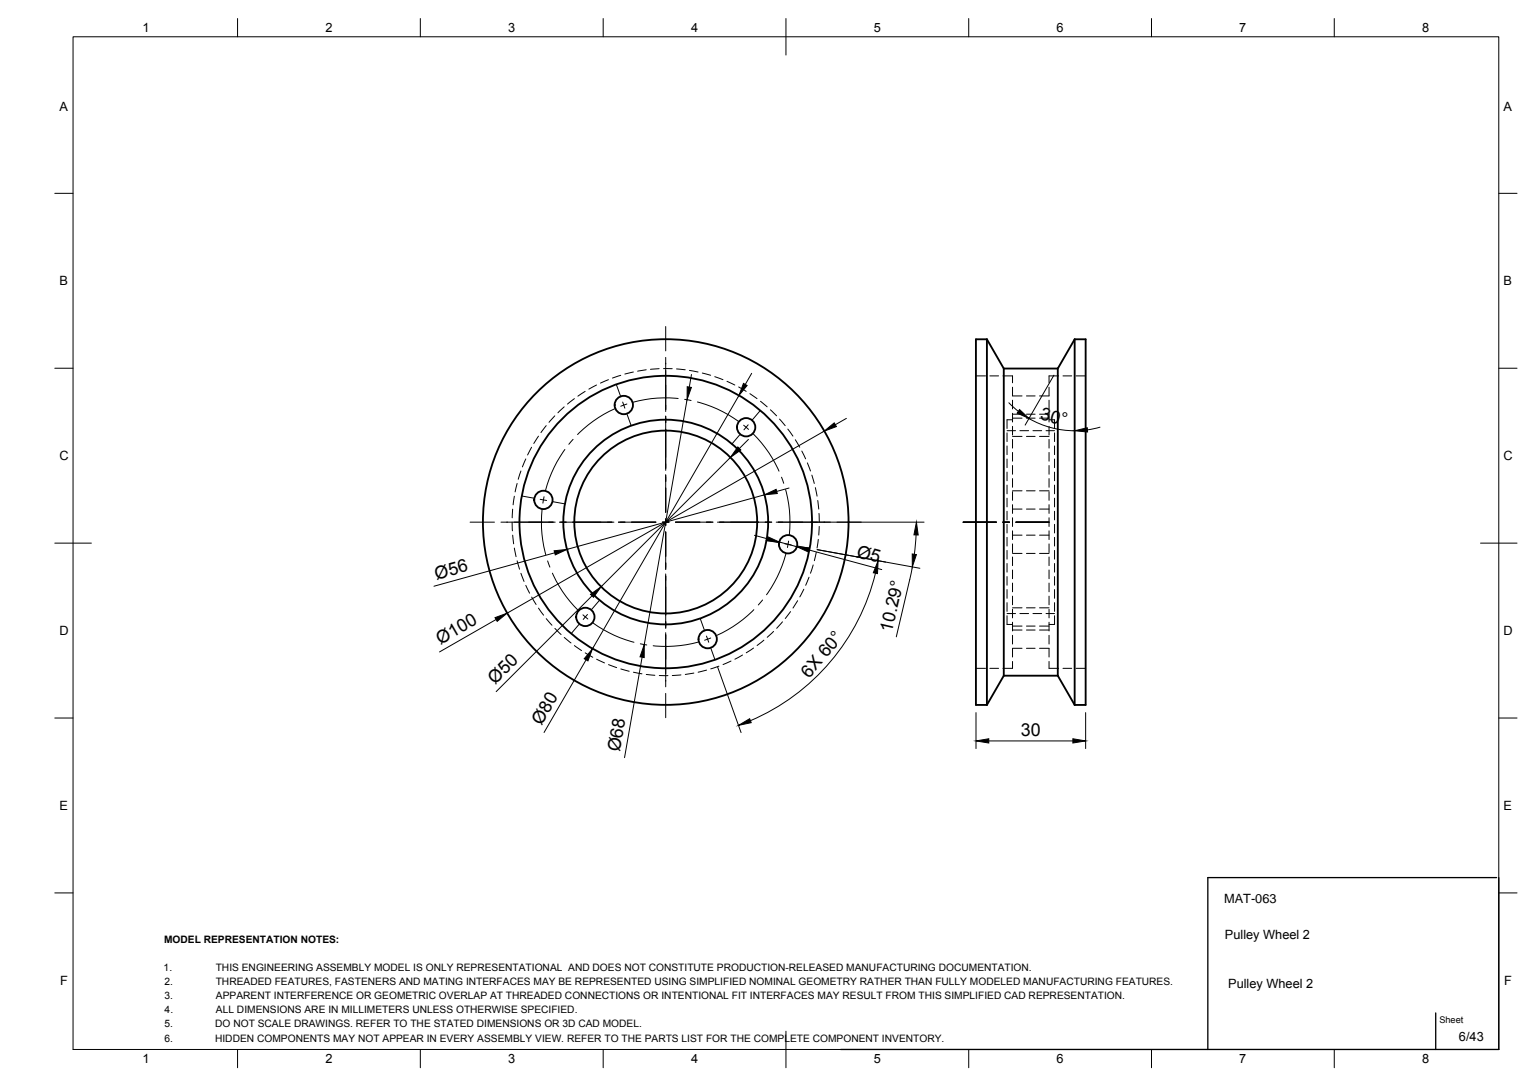
ISO-10303-21;
HEADER;
/* Generated by software containing ST-Developer
 * from STEP Tools, Inc. (www.steptools.com) 
 */

FILE_DESCRIPTION(
/* description */ (''),
/* implementation_level */ '2;1');

FILE_NAME(
/* name */ 'Pulley Wheel 2.step',
/* time_stamp */ '2026-10-24T09:43:01-07:00',
/* author */ (''),
/* organization */ (''),
/* preprocessor_version */ 'ST-DEVELOPER v20.2',
/* originating_system */ 'Autodesk Translation Framework v15.15.0.0',
/* authorisation */ '');

FILE_SCHEMA (('AUTOMOTIVE_DESIGN { 1 0 10303 214 3 1 1 }'));
ENDSEC;

DATA;
#10=MECHANICAL_DESIGN_GEOMETRIC_PRESENTATION_REPRESENTATION('',(#276),#11112);
#210=SHAPE_REPRESENTATION_RELATIONSHIP('SRR','None',#11233,#243);
#243=ADVANCED_BREP_SHAPE_REPRESENTATION('',(#309),#11078);
#276=STYLED_ITEM('',(#11424),#309);
#309=MANIFOLD_SOLID_BREP('Pulley Wheel 2',#6013);
#365=FACE_BOUND('',#1131,.T.);
#366=FACE_BOUND('',#1133,.T.);
#367=FACE_BOUND('',#1137,.T.);
#368=FACE_BOUND('',#1138,.T.);
#369=FACE_BOUND('',#1139,.T.);
#370=FACE_BOUND('',#1140,.T.);
#371=FACE_BOUND('',#1141,.T.);
#372=FACE_BOUND('',#1142,.T.);
#373=FACE_BOUND('',#1143,.T.);
#374=FACE_BOUND('',#1145,.T.);
#375=FACE_BOUND('',#1146,.T.);
#376=FACE_BOUND('',#1147,.T.);
#377=FACE_BOUND('',#1148,.T.);
#378=FACE_BOUND('',#1149,.T.);
#379=FACE_BOUND('',#1150,.T.);
#380=FACE_BOUND('',#1151,.T.);
#381=FACE_BOUND('',#1161,.T.);
#382=FACE_BOUND('',#1163,.T.);
#510=PLANE('',#6593);
#511=PLANE('',#6595);
#512=PLANE('',#6601);
#513=PLANE('',#6609);
#514=PLANE('',#6627);
#515=PLANE('',#6629);
#667=CONICAL_SURFACE('',#6584,1.,1.04719756558882);
#668=CONICAL_SURFACE('',#6586,1.,1.04719756558882);
#735=FACE_OUTER_BOUND('',#1125,.T.);
#736=FACE_OUTER_BOUND('',#1126,.T.);
#737=FACE_OUTER_BOUND('',#1127,.T.);
#738=FACE_OUTER_BOUND('',#1128,.T.);
#739=FACE_OUTER_BOUND('',#1129,.T.);
#740=FACE_OUTER_BOUND('',#1130,.T.);
#741=FACE_OUTER_BOUND('',#1132,.T.);
#742=FACE_OUTER_BOUND('',#1134,.T.);
#743=FACE_OUTER_BOUND('',#1135,.T.);
#744=FACE_OUTER_BOUND('',#1136,.T.);
#745=FACE_OUTER_BOUND('',#1144,.T.);
#746=FACE_OUTER_BOUND('',#1152,.T.);
#747=FACE_OUTER_BOUND('',#1153,.T.);
#748=FACE_OUTER_BOUND('',#1154,.T.);
#749=FACE_OUTER_BOUND('',#1155,.T.);
#750=FACE_OUTER_BOUND('',#1156,.T.);
#751=FACE_OUTER_BOUND('',#1157,.T.);
#752=FACE_OUTER_BOUND('',#1158,.T.);
#753=FACE_OUTER_BOUND('',#1159,.T.);
#754=FACE_OUTER_BOUND('',#1160,.T.);
#755=FACE_OUTER_BOUND('',#1162,.T.);
#756=FACE_OUTER_BOUND('',#1164,.T.);
#1125=EDGE_LOOP('',(#4221,#4222,#4223,#4224,#4225));
#1126=EDGE_LOOP('',(#4226,#4227,#4228,#4229,#4230));
#1127=EDGE_LOOP('',(#4231,#4232,#4233,#4234,#4235));
#1128=EDGE_LOOP('',(#4236,#4237,#4238,#4239));
#1129=EDGE_LOOP('',(#4240,#4241,#4242,#4243,#4244));
#1130=EDGE_LOOP('',(#4245));
#1131=EDGE_LOOP('',(#4246));
#1132=EDGE_LOOP('',(#4247));
#1133=EDGE_LOOP('',(#4248));
#1134=EDGE_LOOP('',(#4249,#4250,#4251,#4252));
#1135=EDGE_LOOP('',(#4253,#4254,#4255,#4256));
#1136=EDGE_LOOP('',(#4257));
#1137=EDGE_LOOP('',(#4258));
#1138=EDGE_LOOP('',(#4259));
#1139=EDGE_LOOP('',(#4260));
#1140=EDGE_LOOP('',(#4261));
#1141=EDGE_LOOP('',(#4262));
#1142=EDGE_LOOP('',(#4263));
#1143=EDGE_LOOP('',(#4264));
#1144=EDGE_LOOP('',(#4265));
#1145=EDGE_LOOP('',(#4266));
#1146=EDGE_LOOP('',(#4267));
#1147=EDGE_LOOP('',(#4268));
#1148=EDGE_LOOP('',(#4269));
#1149=EDGE_LOOP('',(#4270));
#1150=EDGE_LOOP('',(#4271));
#1151=EDGE_LOOP('',(#4272));
#1152=EDGE_LOOP('',(#4273,#4274,#4275,#4276));
#1153=EDGE_LOOP('',(#4277,#4278,#4279,#4280));
#1154=EDGE_LOOP('',(#4281,#4282,#4283,#4284));
#1155=EDGE_LOOP('',(#4285,#4286,#4287,#4288));
#1156=EDGE_LOOP('',(#4289,#4290,#4291,#4292));
#1157=EDGE_LOOP('',(#4293,#4294,#4295,#4296));
#1158=EDGE_LOOP('',(#4297,#4298,#4299,#4300));
#1159=EDGE_LOOP('',(#4301,#4302,#4303,#4304));
#1160=EDGE_LOOP('',(#4305));
#1161=EDGE_LOOP('',(#4306));
#1162=EDGE_LOOP('',(#4307));
#1163=EDGE_LOOP('',(#4308));
#1164=EDGE_LOOP('',(#4309,#4310,#4311,#4312));
#1586=LINE('',#9616,#1945);
#1587=LINE('',#9623,#1946);
#1588=LINE('',#9628,#1947);
#1589=LINE('',#9633,#1948);
#1590=LINE('',#9636,#1949);
#1591=LINE('',#9647,#1950);
#1592=LINE('',#9650,#1951);
#1593=LINE('',#9685,#1952);
#1594=LINE('',#9687,#1953);
#1595=LINE('',#9689,#1954);
#1596=LINE('',#9691,#1955);
#1597=LINE('',#9693,#1956);
#1598=LINE('',#9695,#1957);
#1599=LINE('',#9697,#1958);
#1600=LINE('',#9700,#1959);
#1601=LINE('',#9709,#1960);
#1945=VECTOR('',#7638,0.042);
#1946=VECTOR('',#7647,1.);
#1947=VECTOR('',#7652,1.);
#1948=VECTOR('',#7659,0.05);
#1949=VECTOR('',#7662,0.05);
#1950=VECTOR('',#7677,0.04);
#1951=VECTOR('',#7680,0.04);
#1952=VECTOR('',#7719,0.028);
#1953=VECTOR('',#7722,0.0025);
#1954=VECTOR('',#7725,0.0025);
#1955=VECTOR('',#7728,0.0025);
#1956=VECTOR('',#7731,0.0025);
#1957=VECTOR('',#7734,0.0025);
#1958=VECTOR('',#7737,0.0025);
#1959=VECTOR('',#7740,0.028);
#1960=VECTOR('',#7753,0.025);
#2382=CIRCLE('',#6581,0.042);
#2383=CIRCLE('',#6582,0.042);
#2384=CIRCLE('',#6583,0.042);
#2385=CIRCLE('',#6585,0.05);
#2386=CIRCLE('',#6587,0.05);
#2387=CIRCLE('',#6588,0.05);
#2388=CIRCLE('',#6590,0.05);
#2389=CIRCLE('',#6592,0.05);
#2390=CIRCLE('',#6594,0.04);
#2391=CIRCLE('',#6596,0.04);
#2392=CIRCLE('',#6598,0.04);
#2393=CIRCLE('',#6600,0.04);
#2394=CIRCLE('',#6602,0.0025);
#2395=CIRCLE('',#6603,0.0025);
#2396=CIRCLE('',#6604,0.0025);
#2397=CIRCLE('',#6605,0.0025);
#2398=CIRCLE('',#6606,0.0025);
#2399=CIRCLE('',#6607,0.0025);
#2400=CIRCLE('',#6608,0.028);
#2401=CIRCLE('',#6610,0.0025);
#2402=CIRCLE('',#6611,0.0025);
#2403=CIRCLE('',#6612,0.0025);
#2404=CIRCLE('',#6613,0.0025);
#2405=CIRCLE('',#6614,0.0025);
#2406=CIRCLE('',#6615,0.0025);
#2407=CIRCLE('',#6616,0.028);
#2408=CIRCLE('',#6618,0.028);
#2409=CIRCLE('',#6626,0.028);
#2410=CIRCLE('',#6628,0.025);
#2411=CIRCLE('',#6630,0.025);
#2768=VERTEX_POINT('',#9613);
#2769=VERTEX_POINT('',#9615);
#2770=VERTEX_POINT('',#9617);
#2771=VERTEX_POINT('',#9621);
#2772=VERTEX_POINT('',#9625);
#2773=VERTEX_POINT('',#9626);
#2774=VERTEX_POINT('',#9631);
#2775=VERTEX_POINT('',#9635);
#2776=VERTEX_POINT('',#9639);
#2777=VERTEX_POINT('',#9642);
#2778=VERTEX_POINT('',#9645);
#2779=VERTEX_POINT('',#9649);
#2780=VERTEX_POINT('',#9653);
#2781=VERTEX_POINT('',#9655);
#2782=VERTEX_POINT('',#9657);
#2783=VERTEX_POINT('',#9659);
#2784=VERTEX_POINT('',#9661);
#2785=VERTEX_POINT('',#9663);
#2786=VERTEX_POINT('',#9665);
#2787=VERTEX_POINT('',#9668);
#2788=VERTEX_POINT('',#9670);
#2789=VERTEX_POINT('',#9672);
#2790=VERTEX_POINT('',#9674);
#2791=VERTEX_POINT('',#9676);
#2792=VERTEX_POINT('',#9678);
#2793=VERTEX_POINT('',#9680);
#2794=VERTEX_POINT('',#9683);
#2795=VERTEX_POINT('',#9699);
#2796=VERTEX_POINT('',#9703);
#2797=VERTEX_POINT('',#9706);
#3314=EDGE_CURVE('',#2768,#2768,#2382,.F.);
#3315=EDGE_CURVE('',#2768,#2769,#1586,.T.);
#3316=EDGE_CURVE('',#2769,#2770,#2383,.F.);
#3317=EDGE_CURVE('',#2770,#2769,#2384,.F.);
#3318=EDGE_CURVE('',#2771,#2771,#2385,.F.);
#3319=EDGE_CURVE('',#2771,#2770,#1587,.T.);
#3320=EDGE_CURVE('',#2772,#2773,#2386,.F.);
#3321=EDGE_CURVE('',#2773,#2768,#1588,.T.);
#3322=EDGE_CURVE('',#2773,#2772,#2387,.F.);
#3323=EDGE_CURVE('',#2774,#2774,#2388,.F.);
#3324=EDGE_CURVE('',#2774,#2771,#1589,.T.);
#3325=EDGE_CURVE('',#2772,#2775,#1590,.T.);
#3326=EDGE_CURVE('',#2775,#2775,#2389,.T.);
#3327=EDGE_CURVE('',#2776,#2776,#2390,.T.);
#3328=EDGE_CURVE('',#2777,#2777,#2391,.T.);
#3329=EDGE_CURVE('',#2778,#2778,#2392,.T.);
#3330=EDGE_CURVE('',#2778,#2776,#1591,.T.);
#3331=EDGE_CURVE('',#2777,#2779,#1592,.T.);
#3332=EDGE_CURVE('',#2779,#2779,#2393,.F.);
#3333=EDGE_CURVE('',#2780,#2780,#2394,.F.);
#3334=EDGE_CURVE('',#2781,#2781,#2395,.F.);
#3335=EDGE_CURVE('',#2782,#2782,#2396,.F.);
#3336=EDGE_CURVE('',#2783,#2783,#2397,.F.);
#3337=EDGE_CURVE('',#2784,#2784,#2398,.F.);
#3338=EDGE_CURVE('',#2785,#2785,#2399,.F.);
#3339=EDGE_CURVE('',#2786,#2786,#2400,.T.);
#3340=EDGE_CURVE('',#2787,#2787,#2401,.F.);
#3341=EDGE_CURVE('',#2788,#2788,#2402,.F.);
#3342=EDGE_CURVE('',#2789,#2789,#2403,.F.);
#3343=EDGE_CURVE('',#2790,#2790,#2404,.F.);
#3344=EDGE_CURVE('',#2791,#2791,#2405,.F.);
#3345=EDGE_CURVE('',#2792,#2792,#2406,.F.);
#3346=EDGE_CURVE('',#2793,#2793,#2407,.T.);
#3347=EDGE_CURVE('',#2794,#2794,#2408,.F.);
#3348=EDGE_CURVE('',#2794,#2786,#1593,.T.);
#3349=EDGE_CURVE('',#2785,#2792,#1594,.T.);
#3350=EDGE_CURVE('',#2784,#2791,#1595,.T.);
#3351=EDGE_CURVE('',#2783,#2790,#1596,.T.);
#3352=EDGE_CURVE('',#2782,#2789,#1597,.T.);
#3353=EDGE_CURVE('',#2781,#2788,#1598,.T.);
#3354=EDGE_CURVE('',#2780,#2787,#1599,.T.);
#3355=EDGE_CURVE('',#2793,#2795,#1600,.T.);
#3356=EDGE_CURVE('',#2795,#2795,#2409,.T.);
#3357=EDGE_CURVE('',#2796,#2796,#2410,.T.);
#3358=EDGE_CURVE('',#2797,#2797,#2411,.T.);
#3359=EDGE_CURVE('',#2797,#2796,#1601,.T.);
#4221=ORIENTED_EDGE('',*,*,#3314,.T.);
#4222=ORIENTED_EDGE('',*,*,#3315,.T.);
#4223=ORIENTED_EDGE('',*,*,#3316,.T.);
#4224=ORIENTED_EDGE('',*,*,#3317,.T.);
#4225=ORIENTED_EDGE('',*,*,#3315,.F.);
#4226=ORIENTED_EDGE('',*,*,#3318,.T.);
#4227=ORIENTED_EDGE('',*,*,#3319,.T.);
#4228=ORIENTED_EDGE('',*,*,#3316,.F.);
#4229=ORIENTED_EDGE('',*,*,#3317,.F.);
#4230=ORIENTED_EDGE('',*,*,#3319,.F.);
#4231=ORIENTED_EDGE('',*,*,#3320,.T.);
#4232=ORIENTED_EDGE('',*,*,#3321,.T.);
#4233=ORIENTED_EDGE('',*,*,#3314,.F.);
#4234=ORIENTED_EDGE('',*,*,#3321,.F.);
#4235=ORIENTED_EDGE('',*,*,#3322,.T.);
#4236=ORIENTED_EDGE('',*,*,#3323,.T.);
#4237=ORIENTED_EDGE('',*,*,#3324,.T.);
#4238=ORIENTED_EDGE('',*,*,#3318,.F.);
#4239=ORIENTED_EDGE('',*,*,#3324,.F.);
#4240=ORIENTED_EDGE('',*,*,#3320,.F.);
#4241=ORIENTED_EDGE('',*,*,#3325,.T.);
#4242=ORIENTED_EDGE('',*,*,#3326,.T.);
#4243=ORIENTED_EDGE('',*,*,#3325,.F.);
#4244=ORIENTED_EDGE('',*,*,#3322,.F.);
#4245=ORIENTED_EDGE('',*,*,#3323,.F.);
#4246=ORIENTED_EDGE('',*,*,#3327,.F.);
#4247=ORIENTED_EDGE('',*,*,#3326,.F.);
#4248=ORIENTED_EDGE('',*,*,#3328,.T.);
#4249=ORIENTED_EDGE('',*,*,#3329,.F.);
#4250=ORIENTED_EDGE('',*,*,#3330,.T.);
#4251=ORIENTED_EDGE('',*,*,#3327,.T.);
#4252=ORIENTED_EDGE('',*,*,#3330,.F.);
#4253=ORIENTED_EDGE('',*,*,#3328,.F.);
#4254=ORIENTED_EDGE('',*,*,#3331,.T.);
#4255=ORIENTED_EDGE('',*,*,#3332,.F.);
#4256=ORIENTED_EDGE('',*,*,#3331,.F.);
#4257=ORIENTED_EDGE('',*,*,#3329,.T.);
#4258=ORIENTED_EDGE('',*,*,#3333,.F.);
#4259=ORIENTED_EDGE('',*,*,#3334,.F.);
#4260=ORIENTED_EDGE('',*,*,#3335,.F.);
#4261=ORIENTED_EDGE('',*,*,#3336,.F.);
#4262=ORIENTED_EDGE('',*,*,#3337,.F.);
#4263=ORIENTED_EDGE('',*,*,#3338,.F.);
#4264=ORIENTED_EDGE('',*,*,#3339,.F.);
#4265=ORIENTED_EDGE('',*,*,#3332,.T.);
#4266=ORIENTED_EDGE('',*,*,#3340,.T.);
#4267=ORIENTED_EDGE('',*,*,#3341,.T.);
#4268=ORIENTED_EDGE('',*,*,#3342,.T.);
#4269=ORIENTED_EDGE('',*,*,#3343,.T.);
#4270=ORIENTED_EDGE('',*,*,#3344,.T.);
#4271=ORIENTED_EDGE('',*,*,#3345,.T.);
#4272=ORIENTED_EDGE('',*,*,#3346,.T.);
#4273=ORIENTED_EDGE('',*,*,#3347,.T.);
#4274=ORIENTED_EDGE('',*,*,#3348,.T.);
#4275=ORIENTED_EDGE('',*,*,#3339,.T.);
#4276=ORIENTED_EDGE('',*,*,#3348,.F.);
#4277=ORIENTED_EDGE('',*,*,#3338,.T.);
#4278=ORIENTED_EDGE('',*,*,#3349,.T.);
#4279=ORIENTED_EDGE('',*,*,#3345,.F.);
#4280=ORIENTED_EDGE('',*,*,#3349,.F.);
#4281=ORIENTED_EDGE('',*,*,#3337,.T.);
#4282=ORIENTED_EDGE('',*,*,#3350,.T.);
#4283=ORIENTED_EDGE('',*,*,#3344,.F.);
#4284=ORIENTED_EDGE('',*,*,#3350,.F.);
#4285=ORIENTED_EDGE('',*,*,#3336,.T.);
#4286=ORIENTED_EDGE('',*,*,#3351,.T.);
#4287=ORIENTED_EDGE('',*,*,#3343,.F.);
#4288=ORIENTED_EDGE('',*,*,#3351,.F.);
#4289=ORIENTED_EDGE('',*,*,#3335,.T.);
#4290=ORIENTED_EDGE('',*,*,#3352,.T.);
#4291=ORIENTED_EDGE('',*,*,#3342,.F.);
#4292=ORIENTED_EDGE('',*,*,#3352,.F.);
#4293=ORIENTED_EDGE('',*,*,#3334,.T.);
#4294=ORIENTED_EDGE('',*,*,#3353,.T.);
#4295=ORIENTED_EDGE('',*,*,#3341,.F.);
#4296=ORIENTED_EDGE('',*,*,#3353,.F.);
#4297=ORIENTED_EDGE('',*,*,#3333,.T.);
#4298=ORIENTED_EDGE('',*,*,#3354,.T.);
#4299=ORIENTED_EDGE('',*,*,#3340,.F.);
#4300=ORIENTED_EDGE('',*,*,#3354,.F.);
#4301=ORIENTED_EDGE('',*,*,#3346,.F.);
#4302=ORIENTED_EDGE('',*,*,#3355,.T.);
#4303=ORIENTED_EDGE('',*,*,#3356,.T.);
#4304=ORIENTED_EDGE('',*,*,#3355,.F.);
#4305=ORIENTED_EDGE('',*,*,#3347,.F.);
#4306=ORIENTED_EDGE('',*,*,#3357,.F.);
#4307=ORIENTED_EDGE('',*,*,#3356,.F.);
#4308=ORIENTED_EDGE('',*,*,#3358,.T.);
#4309=ORIENTED_EDGE('',*,*,#3358,.F.);
#4310=ORIENTED_EDGE('',*,*,#3359,.T.);
#4311=ORIENTED_EDGE('',*,*,#3357,.T.);
#4312=ORIENTED_EDGE('',*,*,#3359,.F.);
#5525=CYLINDRICAL_SURFACE('',#6580,0.042);
#5526=CYLINDRICAL_SURFACE('',#6589,0.05);
#5527=CYLINDRICAL_SURFACE('',#6591,0.05);
#5528=CYLINDRICAL_SURFACE('',#6597,0.04);
#5529=CYLINDRICAL_SURFACE('',#6599,0.04);
#5530=CYLINDRICAL_SURFACE('',#6617,0.028);
#5531=CYLINDRICAL_SURFACE('',#6619,0.0025);
#5532=CYLINDRICAL_SURFACE('',#6620,0.0025);
#5533=CYLINDRICAL_SURFACE('',#6621,0.0025);
#5534=CYLINDRICAL_SURFACE('',#6622,0.0025);
#5535=CYLINDRICAL_SURFACE('',#6623,0.0025);
#5536=CYLINDRICAL_SURFACE('',#6624,0.0025);
#5537=CYLINDRICAL_SURFACE('',#6625,0.028);
#5538=CYLINDRICAL_SURFACE('',#6631,0.025);
#5708=ADVANCED_FACE('',(#735),#5525,.T.);
#5709=ADVANCED_FACE('',(#736),#667,.T.);
#5710=ADVANCED_FACE('',(#737),#668,.T.);
#5711=ADVANCED_FACE('',(#738),#5526,.T.);
#5712=ADVANCED_FACE('',(#739),#5527,.T.);
#5713=ADVANCED_FACE('',(#740,#365),#510,.F.);
#5714=ADVANCED_FACE('',(#741,#366),#511,.T.);
#5715=ADVANCED_FACE('',(#742),#5528,.F.);
#5716=ADVANCED_FACE('',(#743),#5529,.F.);
#5717=ADVANCED_FACE('',(#744,#367,#368,#369,#370,#371,#372,#373),#512,.F.);
#5718=ADVANCED_FACE('',(#745,#374,#375,#376,#377,#378,#379,#380),#513,.T.);
#5719=ADVANCED_FACE('',(#746),#5530,.T.);
#5720=ADVANCED_FACE('',(#747),#5531,.F.);
#5721=ADVANCED_FACE('',(#748),#5532,.F.);
#5722=ADVANCED_FACE('',(#749),#5533,.F.);
#5723=ADVANCED_FACE('',(#750),#5534,.F.);
#5724=ADVANCED_FACE('',(#751),#5535,.F.);
#5725=ADVANCED_FACE('',(#752),#5536,.F.);
#5726=ADVANCED_FACE('',(#753),#5537,.T.);
#5727=ADVANCED_FACE('',(#754,#381),#514,.F.);
#5728=ADVANCED_FACE('',(#755,#382),#515,.T.);
#5729=ADVANCED_FACE('',(#756),#5538,.F.);
#6013=CLOSED_SHELL('',(#5708,#5709,#5710,#5711,#5712,#5713,#5714,#5715,
#5716,#5717,#5718,#5719,#5720,#5721,#5722,#5723,#5724,#5725,#5726,#5727,
#5728,#5729));
#6579=AXIS2_PLACEMENT_3D('',#9611,#7632,#7633);
#6580=AXIS2_PLACEMENT_3D('',#9612,#7634,#7635);
#6581=AXIS2_PLACEMENT_3D('',#9614,#7636,#7637);
#6582=AXIS2_PLACEMENT_3D('',#9618,#7639,#7640);
#6583=AXIS2_PLACEMENT_3D('',#9619,#7641,#7642);
#6584=AXIS2_PLACEMENT_3D('',#9620,#7643,#7644);
#6585=AXIS2_PLACEMENT_3D('',#9622,#7645,#7646);
#6586=AXIS2_PLACEMENT_3D('',#9624,#7648,#7649);
#6587=AXIS2_PLACEMENT_3D('',#9627,#7650,#7651);
#6588=AXIS2_PLACEMENT_3D('',#9629,#7653,#7654);
#6589=AXIS2_PLACEMENT_3D('',#9630,#7655,#7656);
#6590=AXIS2_PLACEMENT_3D('',#9632,#7657,#7658);
#6591=AXIS2_PLACEMENT_3D('',#9634,#7660,#7661);
#6592=AXIS2_PLACEMENT_3D('',#9637,#7663,#7664);
#6593=AXIS2_PLACEMENT_3D('',#9638,#7665,#7666);
#6594=AXIS2_PLACEMENT_3D('',#9640,#7667,#7668);
#6595=AXIS2_PLACEMENT_3D('',#9641,#7669,#7670);
#6596=AXIS2_PLACEMENT_3D('',#9643,#7671,#7672);
#6597=AXIS2_PLACEMENT_3D('',#9644,#7673,#7674);
#6598=AXIS2_PLACEMENT_3D('',#9646,#7675,#7676);
#6599=AXIS2_PLACEMENT_3D('',#9648,#7678,#7679);
#6600=AXIS2_PLACEMENT_3D('',#9651,#7681,#7682);
#6601=AXIS2_PLACEMENT_3D('',#9652,#7683,#7684);
#6602=AXIS2_PLACEMENT_3D('',#9654,#7685,#7686);
#6603=AXIS2_PLACEMENT_3D('',#9656,#7687,#7688);
#6604=AXIS2_PLACEMENT_3D('',#9658,#7689,#7690);
#6605=AXIS2_PLACEMENT_3D('',#9660,#7691,#7692);
#6606=AXIS2_PLACEMENT_3D('',#9662,#7693,#7694);
#6607=AXIS2_PLACEMENT_3D('',#9664,#7695,#7696);
#6608=AXIS2_PLACEMENT_3D('',#9666,#7697,#7698);
#6609=AXIS2_PLACEMENT_3D('',#9667,#7699,#7700);
#6610=AXIS2_PLACEMENT_3D('',#9669,#7701,#7702);
#6611=AXIS2_PLACEMENT_3D('',#9671,#7703,#7704);
#6612=AXIS2_PLACEMENT_3D('',#9673,#7705,#7706);
#6613=AXIS2_PLACEMENT_3D('',#9675,#7707,#7708);
#6614=AXIS2_PLACEMENT_3D('',#9677,#7709,#7710);
#6615=AXIS2_PLACEMENT_3D('',#9679,#7711,#7712);
#6616=AXIS2_PLACEMENT_3D('',#9681,#7713,#7714);
#6617=AXIS2_PLACEMENT_3D('',#9682,#7715,#7716);
#6618=AXIS2_PLACEMENT_3D('',#9684,#7717,#7718);
#6619=AXIS2_PLACEMENT_3D('',#9686,#7720,#7721);
#6620=AXIS2_PLACEMENT_3D('',#9688,#7723,#7724);
#6621=AXIS2_PLACEMENT_3D('',#9690,#7726,#7727);
#6622=AXIS2_PLACEMENT_3D('',#9692,#7729,#7730);
#6623=AXIS2_PLACEMENT_3D('',#9694,#7732,#7733);
#6624=AXIS2_PLACEMENT_3D('',#9696,#7735,#7736);
#6625=AXIS2_PLACEMENT_3D('',#9698,#7738,#7739);
#6626=AXIS2_PLACEMENT_3D('',#9701,#7741,#7742);
#6627=AXIS2_PLACEMENT_3D('',#9702,#7743,#7744);
#6628=AXIS2_PLACEMENT_3D('',#9704,#7745,#7746);
#6629=AXIS2_PLACEMENT_3D('',#9705,#7747,#7748);
#6630=AXIS2_PLACEMENT_3D('',#9707,#7749,#7750);
#6631=AXIS2_PLACEMENT_3D('',#9708,#7751,#7752);
#7632=DIRECTION('axis',(0.,0.,1.));
#7633=DIRECTION('refdir',(1.,0.,0.));
#7634=DIRECTION('center_axis',(4.13029399042097E-17,0.,1.));
#7635=DIRECTION('ref_axis',(1.,0.,-4.13029399042097E-17));
#7636=DIRECTION('center_axis',(-3.04809470411818E-27,2.64338815530979E-17,
1.));
#7637=DIRECTION('ref_axis',(1.,-4.29586510583046E-10,0.));
#7638=DIRECTION('',(-4.13029399042097E-17,0.,-1.));
#7639=DIRECTION('center_axis',(-5.28677630773884E-17,-1.0843360466812E-26,
-1.));
#7640=DIRECTION('ref_axis',(1.,2.50000086925735E-10,-5.28677630773884E-17));
#7641=DIRECTION('center_axis',(-5.28677630773884E-17,-1.0843360466812E-26,
-1.));
#7642=DIRECTION('ref_axis',(1.,2.50000086925735E-10,-5.28677630773884E-17));
#7643=DIRECTION('center_axis',(-1.70140119462979E-16,0.,-1.));
#7644=DIRECTION('ref_axis',(-1.,0.,1.70140119462979E-16));
#7645=DIRECTION('center_axis',(-9.76996261870523E-16,-9.7699626151362E-16,
-1.));
#7646=DIRECTION('ref_axis',(1.,-1.60206417040051E-10,-9.76996261670138E-16));
#7647=DIRECTION('',(-0.86602541098055,1.0605752475376E-16,0.49999998753597));
#7648=DIRECTION('center_axis',(1.70140119462979E-16,0.,1.));
#7649=DIRECTION('ref_axis',(1.,0.,-1.70140119462979E-16));
#7650=DIRECTION('center_axis',(0.,0.,1.));
#7651=DIRECTION('ref_axis',(-1.,-1.60206710118277E-10,0.));
#7652=DIRECTION('',(0.86602541098055,1.0605752475376E-16,-0.49999998753597));
#7653=DIRECTION('center_axis',(0.,0.,1.));
#7654=DIRECTION('ref_axis',(-1.,-1.60206710118277E-10,0.));
#7655=DIRECTION('center_axis',(0.,0.,-1.));
#7656=DIRECTION('ref_axis',(-1.,0.,0.));
#7657=DIRECTION('center_axis',(0.,0.,-1.));
#7658=DIRECTION('ref_axis',(-1.,0.,0.));
#7659=DIRECTION('',(0.,0.,1.));
#7660=DIRECTION('center_axis',(0.,0.,-1.));
#7661=DIRECTION('ref_axis',(-1.,0.,0.));
#7662=DIRECTION('',(0.,0.,1.));
#7663=DIRECTION('center_axis',(0.,0.,-1.));
#7664=DIRECTION('ref_axis',(-1.,0.,0.));
#7665=DIRECTION('center_axis',(2.84990285479818E-18,3.64291930135101E-18,
1.));
#7666=DIRECTION('ref_axis',(0.,-1.,3.64291930135101E-18));
#7667=DIRECTION('center_axis',(-2.16840434497101E-17,0.,-1.));
#7668=DIRECTION('ref_axis',(-1.,0.,2.16840434497101E-17));
#7669=DIRECTION('center_axis',(-2.84990285479818E-18,-3.64291930135101E-18,
1.));
#7670=DIRECTION('ref_axis',(0.,-1.,-3.64291930135101E-18));
#7671=DIRECTION('center_axis',(0.,0.,-1.));
#7672=DIRECTION('ref_axis',(-1.,0.,0.));
#7673=DIRECTION('center_axis',(-2.16840434497101E-17,0.,-1.));
#7674=DIRECTION('ref_axis',(-1.,0.,2.16840434497101E-17));
#7675=DIRECTION('center_axis',(-2.16840434497101E-17,0.,-1.));
#7676=DIRECTION('ref_axis',(-1.,0.,2.16840434497101E-17));
#7677=DIRECTION('',(-2.16840434497101E-17,0.,-1.));
#7678=DIRECTION('center_axis',(0.,0.,-1.));
#7679=DIRECTION('ref_axis',(-1.,0.,0.));
#7680=DIRECTION('',(0.,0.,-1.));
#7681=DIRECTION('center_axis',(0.,0.,-1.));
#7682=DIRECTION('ref_axis',(-1.,0.,0.));
#7683=DIRECTION('center_axis',(-6.27288400105048E-18,-2.92734586715581E-18,
1.));
#7684=DIRECTION('ref_axis',(1.,-1.25733582200228E-51,6.27288400105048E-18));
#7685=DIRECTION('center_axis',(-3.46944695195361E-16,0.,1.));
#7686=DIRECTION('ref_axis',(1.,0.,3.46944695195361E-16));
#7687=DIRECTION('center_axis',(-3.46944695195361E-16,0.,1.));
#7688=DIRECTION('ref_axis',(1.,0.,3.46944695195361E-16));
#7689=DIRECTION('center_axis',(-3.46944695195362E-16,0.,1.));
#7690=DIRECTION('ref_axis',(1.,0.,3.46944695195362E-16));
#7691=DIRECTION('center_axis',(-3.46944695195361E-16,0.,1.));
#7692=DIRECTION('ref_axis',(1.,0.,3.46944695195361E-16));
#7693=DIRECTION('center_axis',(-3.46944695195361E-16,0.,1.));
#7694=DIRECTION('ref_axis',(1.,0.,3.46944695195361E-16));
#7695=DIRECTION('center_axis',(-3.46944695195362E-16,0.,1.));
#7696=DIRECTION('ref_axis',(1.,0.,3.46944695195362E-16));
#7697=DIRECTION('center_axis',(0.,0.,-1.));
#7698=DIRECTION('ref_axis',(-1.,0.,0.));
#7699=DIRECTION('center_axis',(6.27288400105048E-18,2.92734586715581E-18,
1.));
#7700=DIRECTION('ref_axis',(1.,-1.25733582200228E-51,-6.27288400105048E-18));
#7701=DIRECTION('center_axis',(-3.46944695195361E-16,0.,1.));
#7702=DIRECTION('ref_axis',(1.,0.,3.46944695195361E-16));
#7703=DIRECTION('center_axis',(-3.46944695195361E-16,0.,1.));
#7704=DIRECTION('ref_axis',(1.,0.,3.46944695195361E-16));
#7705=DIRECTION('center_axis',(-3.46944695195362E-16,0.,1.));
#7706=DIRECTION('ref_axis',(1.,0.,3.46944695195362E-16));
#7707=DIRECTION('center_axis',(-3.46944695195361E-16,0.,1.));
#7708=DIRECTION('ref_axis',(1.,0.,3.46944695195361E-16));
#7709=DIRECTION('center_axis',(-3.46944695195361E-16,0.,1.));
#7710=DIRECTION('ref_axis',(1.,0.,3.46944695195361E-16));
#7711=DIRECTION('center_axis',(-3.46944695195362E-16,0.,1.));
#7712=DIRECTION('ref_axis',(1.,0.,3.46944695195362E-16));
#7713=DIRECTION('center_axis',(0.,0.,-1.));
#7714=DIRECTION('ref_axis',(-1.,0.,0.));
#7715=DIRECTION('center_axis',(0.,0.,-1.));
#7716=DIRECTION('ref_axis',(-1.,0.,0.));
#7717=DIRECTION('center_axis',(0.,0.,-1.));
#7718=DIRECTION('ref_axis',(-1.,0.,0.));
#7719=DIRECTION('',(0.,0.,1.));
#7720=DIRECTION('center_axis',(-3.46944695195362E-16,0.,1.));
#7721=DIRECTION('ref_axis',(1.,0.,3.46944695195362E-16));
#7722=DIRECTION('',(-3.46944695195362E-16,0.,1.));
#7723=DIRECTION('center_axis',(-3.46944695195361E-16,0.,1.));
#7724=DIRECTION('ref_axis',(1.,0.,3.46944695195361E-16));
#7725=DIRECTION('',(-3.46944695195361E-16,0.,1.));
#7726=DIRECTION('center_axis',(-3.46944695195361E-16,0.,1.));
#7727=DIRECTION('ref_axis',(1.,0.,3.46944695195361E-16));
#7728=DIRECTION('',(-3.46944695195361E-16,0.,1.));
#7729=DIRECTION('center_axis',(-3.46944695195362E-16,0.,1.));
#7730=DIRECTION('ref_axis',(1.,0.,3.46944695195362E-16));
#7731=DIRECTION('',(-3.46944695195362E-16,0.,1.));
#7732=DIRECTION('center_axis',(-3.46944695195361E-16,0.,1.));
#7733=DIRECTION('ref_axis',(1.,0.,3.46944695195361E-16));
#7734=DIRECTION('',(-3.46944695195361E-16,0.,1.));
#7735=DIRECTION('center_axis',(-3.46944695195361E-16,0.,1.));
#7736=DIRECTION('ref_axis',(1.,0.,3.46944695195361E-16));
#7737=DIRECTION('',(-3.46944695195361E-16,0.,1.));
#7738=DIRECTION('center_axis',(0.,0.,-1.));
#7739=DIRECTION('ref_axis',(-1.,0.,0.));
#7740=DIRECTION('',(0.,0.,1.));
#7741=DIRECTION('center_axis',(0.,0.,-1.));
#7742=DIRECTION('ref_axis',(-1.,0.,0.));
#7743=DIRECTION('center_axis',(-6.39458016332861E-18,-1.10411609048463E-17,
1.));
#7744=DIRECTION('ref_axis',(0.,-1.,-1.10411609048463E-17));
#7745=DIRECTION('center_axis',(0.,0.,-1.));
#7746=DIRECTION('ref_axis',(-1.,0.,0.));
#7747=DIRECTION('center_axis',(6.39458016332861E-18,1.10411609048463E-17,
1.));
#7748=DIRECTION('ref_axis',(0.,-1.,1.10411609048463E-17));
#7749=DIRECTION('center_axis',(0.,0.,-1.));
#7750=DIRECTION('ref_axis',(-1.,0.,0.));
#7751=DIRECTION('center_axis',(0.,0.,-1.));
#7752=DIRECTION('ref_axis',(-1.,0.,0.));
#7753=DIRECTION('',(0.,0.,-1.));
#9611=CARTESIAN_POINT('',(0.,0.,0.));
#9612=CARTESIAN_POINT('Origin',(-5.74005956283549E-52,0.,0.015));
#9613=CARTESIAN_POINT('',(-0.042,-1.9853686361416E-11,0.007381198));
#9614=CARTESIAN_POINT('Origin',(-2.66453525910038E-17,5.09119415777057E-18,
0.007381198));
#9615=CARTESIAN_POINT('',(-0.042,-1.54820701770975E-11,-0.007381198));
#9616=CARTESIAN_POINT('',(-0.042,-5.14351655641888E-18,0.015));
#9617=CARTESIAN_POINT('',(0.0419999999999985,-5.1435165564187E-18,-0.00738119800000199));
#9618=CARTESIAN_POINT('Origin',(-8.88178419700125E-18,-5.73557577313579E-18,
-0.007381198));
#9619=CARTESIAN_POINT('Origin',(-8.88178419700125E-18,-5.73557577313579E-18,
-0.007381198));
#9620=CARTESIAN_POINT('Origin',(-2.64244881468667E-16,0.,-0.560482737499999));
#9621=CARTESIAN_POINT('',(0.0499999999999997,-6.12323399573673E-18,-0.0120000000000027));
#9622=CARTESIAN_POINT('Origin',(8.88178419700125E-18,1.23918456012259E-18,
-0.012000000000002));
#9623=CARTESIAN_POINT('',(1.,-1.22464679914735E-16,-0.5604827375));
#9624=CARTESIAN_POINT('Origin',(2.63459037944631E-16,0.,0.560482737500119));
#9625=CARTESIAN_POINT('',(0.05,-2.05102985990085E-11,0.0120000000000921));
#9626=CARTESIAN_POINT('',(-0.0499999999999868,-6.12323399573515E-18,0.0120000000001151));
#9627=CARTESIAN_POINT('Origin',(1.77635683940025E-17,-6.31136467490802E-18,
0.0120000000000921));
#9628=CARTESIAN_POINT('',(-1.,-1.22464679914735E-16,0.560482737500119));
#9629=CARTESIAN_POINT('Origin',(1.77635683940025E-17,-6.31136467490802E-18,
0.0120000000000921));
#9630=CARTESIAN_POINT('Origin',(0.,0.,0.015));
#9631=CARTESIAN_POINT('',(0.05,-6.12323399573677E-18,-0.015));
#9632=CARTESIAN_POINT('Origin',(0.,0.,-0.015));
#9633=CARTESIAN_POINT('',(0.05,-6.12323399573677E-18,0.015));
#9634=CARTESIAN_POINT('Origin',(0.,0.,0.015));
#9635=CARTESIAN_POINT('',(0.05,-6.12323399573677E-18,0.015));
#9636=CARTESIAN_POINT('',(0.05,-6.12323399573677E-18,0.015));
#9637=CARTESIAN_POINT('Origin',(0.,0.,0.015));
#9638=CARTESIAN_POINT('Origin',(5.79397640976254E-18,1.73472347597681E-19,
-0.015));
#9639=CARTESIAN_POINT('',(0.04,-4.89858719658941E-18,-0.015));
#9640=CARTESIAN_POINT('Origin',(-6.50521303491303E-19,0.,-0.015));
#9641=CARTESIAN_POINT('Origin',(5.79397640976254E-18,1.73472347597681E-19,
0.015));
#9642=CARTESIAN_POINT('',(0.04,-4.89858719658941E-18,0.015));
#9643=CARTESIAN_POINT('Origin',(0.,0.,0.015));
#9644=CARTESIAN_POINT('Origin',(1.85684700327654E-52,0.,0.015));
#9645=CARTESIAN_POINT('',(0.04,-4.89858719658941E-18,-0.005));
#9646=CARTESIAN_POINT('Origin',(-4.33680868994202E-19,0.,-0.005));
#9647=CARTESIAN_POINT('',(0.04,-4.89858719658941E-18,0.015));
#9648=CARTESIAN_POINT('Origin',(0.,0.,0.015));
#9649=CARTESIAN_POINT('',(0.04,-4.89858719658941E-18,0.005));
#9650=CARTESIAN_POINT('',(0.04,-4.89858719658941E-18,0.015));
#9651=CARTESIAN_POINT('Origin',(0.,0.,0.005));
#9652=CARTESIAN_POINT('Origin',(3.17454396103755E-18,1.73472347597681E-20,
-0.005));
#9653=CARTESIAN_POINT('',(0.026944864,0.017,-0.005));
#9654=CARTESIAN_POINT('Origin',(0.029444864,0.017,-0.005));
#9655=CARTESIAN_POINT('',(0.026944864,-0.017,-0.005));
#9656=CARTESIAN_POINT('Origin',(0.029444864,-0.017,-0.005));
#9657=CARTESIAN_POINT('',(-0.0025,-0.034,-0.005));
#9658=CARTESIAN_POINT('Origin',(-3.46944695195361E-18,-0.034,-0.005));
#9659=CARTESIAN_POINT('',(-0.031944864,-0.017,-0.005));
#9660=CARTESIAN_POINT('Origin',(-0.029444864,-0.017,-0.005));
#9661=CARTESIAN_POINT('',(-0.031944864,0.017,-0.005));
#9662=CARTESIAN_POINT('Origin',(-0.029444864,0.017,-0.005));
#9663=CARTESIAN_POINT('',(-0.0025,0.034,-0.005));
#9664=CARTESIAN_POINT('Origin',(-3.46944695195361E-18,0.034,-0.005));
#9665=CARTESIAN_POINT('',(0.028,-3.42901103761259E-18,-0.005));
#9666=CARTESIAN_POINT('Origin',(0.,0.,-0.005));
#9667=CARTESIAN_POINT('Origin',(3.17454396103755E-18,1.73472347597681E-20,
0.005));
#9668=CARTESIAN_POINT('',(0.026944864,0.017,0.005));
#9669=CARTESIAN_POINT('Origin',(0.029444864,0.017,0.005));
#9670=CARTESIAN_POINT('',(0.026944864,-0.017,0.005));
#9671=CARTESIAN_POINT('Origin',(0.029444864,-0.017,0.005));
#9672=CARTESIAN_POINT('',(-0.00250000000000001,-0.034,0.005));
#9673=CARTESIAN_POINT('Origin',(-6.93889390390723E-18,-0.034,0.005));
#9674=CARTESIAN_POINT('',(-0.031944864,-0.017,0.005));
#9675=CARTESIAN_POINT('Origin',(-0.029444864,-0.017,0.005));
#9676=CARTESIAN_POINT('',(-0.031944864,0.017,0.005));
#9677=CARTESIAN_POINT('Origin',(-0.029444864,0.017,0.005));
#9678=CARTESIAN_POINT('',(-0.00250000000000001,0.034,0.005));
#9679=CARTESIAN_POINT('Origin',(-6.93889390390723E-18,0.034,0.005));
#9680=CARTESIAN_POINT('',(0.028,-3.42901103761259E-18,0.005));
#9681=CARTESIAN_POINT('Origin',(0.,0.,0.005));
#9682=CARTESIAN_POINT('Origin',(0.,0.,0.0065));
#9683=CARTESIAN_POINT('',(0.028,-3.42901103761259E-18,-0.0065));
#9684=CARTESIAN_POINT('Origin',(0.,0.,-0.0065));
#9685=CARTESIAN_POINT('',(0.028,-3.42901103761259E-18,0.0065));
#9686=CARTESIAN_POINT('Origin',(-1.44987137336516E-49,0.034,-0.015));
#9687=CARTESIAN_POINT('',(-0.0025,0.034,-0.015));
#9688=CARTESIAN_POINT('Origin',(-0.029444864,0.017,-0.015));
#9689=CARTESIAN_POINT('',(-0.031944864,0.017,-0.015));
#9690=CARTESIAN_POINT('Origin',(-0.029444864,-0.017,-0.015));
#9691=CARTESIAN_POINT('',(-0.031944864,-0.017,-0.015));
#9692=CARTESIAN_POINT('Origin',(-1.44987137336516E-49,-0.034,-0.015));
#9693=CARTESIAN_POINT('',(-0.0025,-0.034,-0.015));
#9694=CARTESIAN_POINT('Origin',(0.029444864,-0.017,-0.015));
#9695=CARTESIAN_POINT('',(0.026944864,-0.017,-0.015));
#9696=CARTESIAN_POINT('Origin',(0.029444864,0.017,-0.015));
#9697=CARTESIAN_POINT('',(0.026944864,0.017,-0.015));
#9698=CARTESIAN_POINT('Origin',(0.,0.,0.0065));
#9699=CARTESIAN_POINT('',(0.028,-3.42901103761259E-18,0.0065));
#9700=CARTESIAN_POINT('',(0.028,-3.42901103761259E-18,0.0065));
#9701=CARTESIAN_POINT('Origin',(0.,0.,0.0065));
#9702=CARTESIAN_POINT('Origin',(-1.21430643318376E-19,-1.12757025938492E-18,
-0.0065));
#9703=CARTESIAN_POINT('',(0.025,-3.06161699786838E-18,-0.0065));
#9704=CARTESIAN_POINT('Origin',(0.,0.,-0.0065));
#9705=CARTESIAN_POINT('Origin',(-1.21430643318376E-19,-1.12757025938492E-18,
0.0065));
#9706=CARTESIAN_POINT('',(0.025,-3.06161699786838E-18,0.0065));
#9707=CARTESIAN_POINT('Origin',(0.,0.,0.0065));
#9708=CARTESIAN_POINT('Origin',(0.,0.,0.0065));
#9709=CARTESIAN_POINT('',(0.025,-3.06161699786838E-18,0.0065));
#11039=UNCERTAINTY_MEASURE_WITH_UNIT(LENGTH_MEASURE(1.E-5),#11113,
'DISTANCE_ACCURACY_VALUE',
'Maximum model space distance between geometric entities at asserted c
onnectivities');
#11073=UNCERTAINTY_MEASURE_WITH_UNIT(LENGTH_MEASURE(1.E-5),#11113,
'DISTANCE_ACCURACY_VALUE',
'Maximum model space distance between geometric entities at asserted c
onnectivities');
#11078=(
GEOMETRIC_REPRESENTATION_CONTEXT(3)
GLOBAL_UNCERTAINTY_ASSIGNED_CONTEXT((#11039))
GLOBAL_UNIT_ASSIGNED_CONTEXT((#11113,#11114,#11115))
REPRESENTATION_CONTEXT('','3D')
);
#11112=(
GEOMETRIC_REPRESENTATION_CONTEXT(3)
GLOBAL_UNCERTAINTY_ASSIGNED_CONTEXT((#11073))
GLOBAL_UNIT_ASSIGNED_CONTEXT((#11113,#11114,#11115))
REPRESENTATION_CONTEXT('','3D')
);
#11113=(
LENGTH_UNIT()
NAMED_UNIT(*)
SI_UNIT($,.METRE.)
);
#11114=(
NAMED_UNIT(*)
PLANE_ANGLE_UNIT()
SI_UNIT($,.RADIAN.)
);
#11115=(
NAMED_UNIT(*)
SI_UNIT($,.STERADIAN.)
SOLID_ANGLE_UNIT()
);
#11120=SHAPE_DEFINITION_REPRESENTATION(#11158,#11233);
#11158=PRODUCT_DEFINITION_SHAPE('',$,#11272);
#11233=SHAPE_REPRESENTATION('',(#6579),#11078);
#11267=PRODUCT_DEFINITION_CONTEXT('part definition',#11383,'design');
#11272=PRODUCT_DEFINITION('Pulley Wheel 2','Pulley Wheel 2',#11310,#11267);
#11310=PRODUCT_DEFINITION_FORMATION('',$,#11389);
#11383=APPLICATION_CONTEXT(
'Core Data for Automotive Mechanical Design Process');
#11384=PRODUCT_CONTEXT('part definition',#11383,'mechanical');
#11389=PRODUCT('Pulley Wheel 2','Pulley Wheel 2',
'pulleywheel__ DE    11841',(#11384));
#11424=PRESENTATION_STYLE_ASSIGNMENT((#11428));
#11428=SURFACE_STYLE_USAGE(.BOTH.,#11432);
#11432=SURFACE_SIDE_STYLE('',(#11436));
#11436=SURFACE_STYLE_FILL_AREA(#11440);
#11440=FILL_AREA_STYLE('Opaque(198,193,188)',(#11444));
#11444=FILL_AREA_STYLE_COLOUR('Opaque(198,193,188)',#11448);
#11448=COLOUR_RGB('Opaque(198,193,188)',0.776470588235294,0.756862745098039,
0.737254901960784);
ENDSEC;
END-ISO-10303-21;
